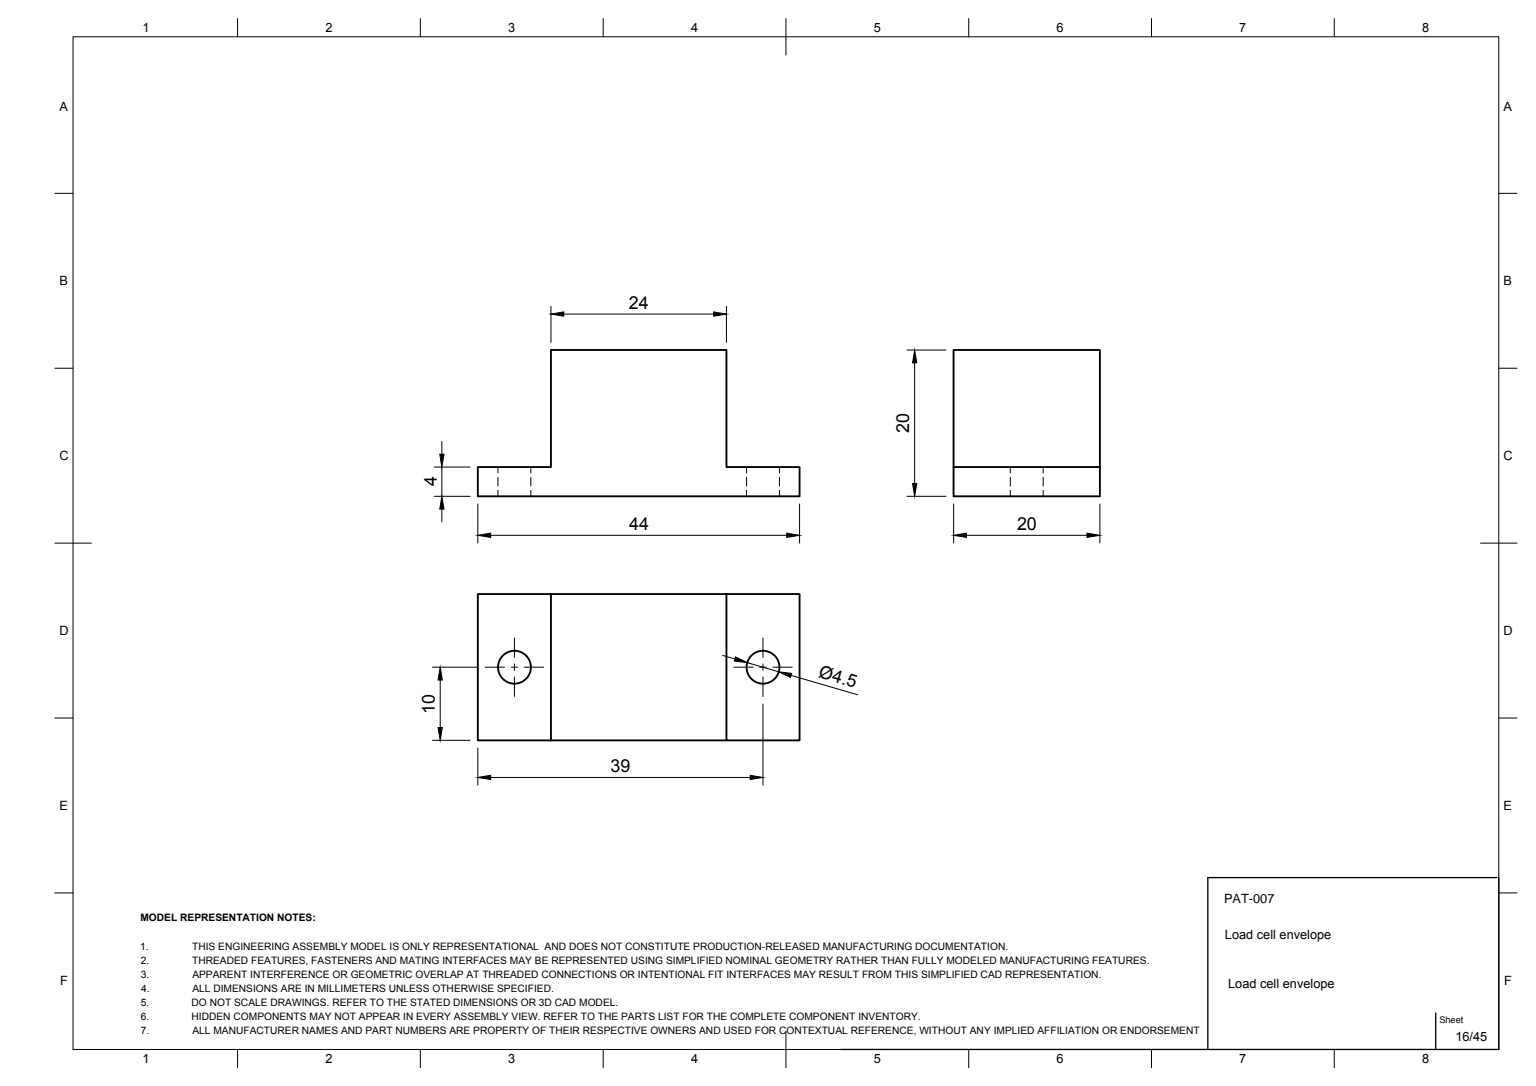
ISO-10303-21;
HEADER;
/* Generated by software containing ST-Developer
 * from STEP Tools, Inc. (www.steptools.com) 
 */

FILE_DESCRIPTION(
/* description */ ('Bearing friction torque test rig'),
/* implementation_level */ '2;1');

FILE_NAME(
/* name */ 'Load cell envelope.step',
/* time_stamp */ '2026-10-28T03:24:04-07:00',
/* author */ (''),
/* organization */ (''),
/* preprocessor_version */ 'ST-DEVELOPER v20.2',
/* originating_system */ 'Autodesk Translation Framework v15.17.0.0',
/* authorisation */ '');

FILE_SCHEMA (('AUTOMOTIVE_DESIGN { 1 0 10303 214 3 1 1 }'));
ENDSEC;

DATA;
#10=MECHANICAL_DESIGN_GEOMETRIC_PRESENTATION_REPRESENTATION('',(#550),#14822);
#472=SHAPE_REPRESENTATION_RELATIONSHIP('SRR','None',#15011,#511);
#511=ADVANCED_BREP_SHAPE_REPRESENTATION('',(#604),#14791);
#550=STYLED_ITEM('',(#15270),#604);
#604=MANIFOLD_SOLID_BREP('Body1',#7666);
#791=FACE_BOUND('',#1849,.T.);
#792=FACE_BOUND('',#1853,.T.);
#793=FACE_BOUND('',#1860,.T.);
#794=FACE_BOUND('',#1861,.T.);
#939=PLANE('',#8507);
#940=PLANE('',#8508);
#941=PLANE('',#8509);
#942=PLANE('',#8510);
#943=PLANE('',#8511);
#944=PLANE('',#8512);
#945=PLANE('',#8513);
#946=PLANE('',#8514);
#947=PLANE('',#8515);
#948=PLANE('',#8516);
#1254=FACE_OUTER_BOUND('',#1846,.T.);
#1255=FACE_OUTER_BOUND('',#1847,.T.);
#1256=FACE_OUTER_BOUND('',#1848,.T.);
#1257=FACE_OUTER_BOUND('',#1850,.T.);
#1258=FACE_OUTER_BOUND('',#1851,.T.);
#1259=FACE_OUTER_BOUND('',#1852,.T.);
#1260=FACE_OUTER_BOUND('',#1854,.T.);
#1261=FACE_OUTER_BOUND('',#1855,.T.);
#1262=FACE_OUTER_BOUND('',#1856,.T.);
#1263=FACE_OUTER_BOUND('',#1857,.T.);
#1264=FACE_OUTER_BOUND('',#1858,.T.);
#1265=FACE_OUTER_BOUND('',#1859,.T.);
#1846=EDGE_LOOP('',(#5844,#5845,#5846,#5847));
#1847=EDGE_LOOP('',(#5848,#5849,#5850,#5851));
#1848=EDGE_LOOP('',(#5852,#5853,#5854,#5855));
#1849=EDGE_LOOP('',(#5856));
#1850=EDGE_LOOP('',(#5857,#5858,#5859,#5860));
#1851=EDGE_LOOP('',(#5861,#5862,#5863,#5864));
#1852=EDGE_LOOP('',(#5865,#5866,#5867,#5868));
#1853=EDGE_LOOP('',(#5869));
#1854=EDGE_LOOP('',(#5870,#5871,#5872,#5873));
#1855=EDGE_LOOP('',(#5874,#5875,#5876,#5877,#5878,#5879,#5880,#5881));
#1856=EDGE_LOOP('',(#5882,#5883,#5884,#5885));
#1857=EDGE_LOOP('',(#5886,#5887,#5888,#5889,#5890,#5891,#5892,#5893));
#1858=EDGE_LOOP('',(#5894,#5895,#5896,#5897));
#1859=EDGE_LOOP('',(#5898,#5899,#5900,#5901));
#1860=EDGE_LOOP('',(#5902));
#1861=EDGE_LOOP('',(#5903));
#2377=LINE('',#12411,#2821);
#2378=LINE('',#12417,#2822);
#2379=LINE('',#12422,#2823);
#2380=LINE('',#12424,#2824);
#2381=LINE('',#12426,#2825);
#2382=LINE('',#12427,#2826);
#2383=LINE('',#12430,#2827);
#2384=LINE('',#12432,#2828);
#2385=LINE('',#12433,#2829);
#2386=LINE('',#12436,#2830);
#2387=LINE('',#12438,#2831);
#2388=LINE('',#12439,#2832);
#2389=LINE('',#12443,#2833);
#2390=LINE('',#12445,#2834);
#2391=LINE('',#12447,#2835);
#2392=LINE('',#12448,#2836);
#2393=LINE('',#12451,#2837);
#2394=LINE('',#12453,#2838);
#2395=LINE('',#12454,#2839);
#2396=LINE('',#12456,#2840);
#2397=LINE('',#12458,#2841);
#2398=LINE('',#12459,#2842);
#2399=LINE('',#12462,#2843);
#2400=LINE('',#12463,#2844);
#2401=LINE('',#12465,#2845);
#2402=LINE('',#12466,#2846);
#2821=VECTOR('',#10046,0.225);
#2822=VECTOR('',#10053,0.225);
#2823=VECTOR('',#10058,1.);
#2824=VECTOR('',#10059,1.);
#2825=VECTOR('',#10060,1.);
#2826=VECTOR('',#10061,1.);
#2827=VECTOR('',#10064,1.);
#2828=VECTOR('',#10065,1.);
#2829=VECTOR('',#10066,1.);
#2830=VECTOR('',#10069,1.);
#2831=VECTOR('',#10070,1.);
#2832=VECTOR('',#10071,1.);
#2833=VECTOR('',#10074,1.);
#2834=VECTOR('',#10075,1.);
#2835=VECTOR('',#10076,1.);
#2836=VECTOR('',#10077,1.);
#2837=VECTOR('',#10080,1.);
#2838=VECTOR('',#10081,1.);
#2839=VECTOR('',#10082,1.);
#2840=VECTOR('',#10085,1.);
#2841=VECTOR('',#10086,1.);
#2842=VECTOR('',#10087,1.);
#2843=VECTOR('',#10090,1.);
#2844=VECTOR('',#10091,1.);
#2845=VECTOR('',#10094,1.);
#2846=VECTOR('',#10095,1.);
#3291=CIRCLE('',#8502,0.225);
#3292=CIRCLE('',#8503,0.225);
#3293=CIRCLE('',#8505,0.225);
#3294=CIRCLE('',#8506,0.225);
#3785=VERTEX_POINT('',#12408);
#3786=VERTEX_POINT('',#12410);
#3787=VERTEX_POINT('',#12414);
#3788=VERTEX_POINT('',#12416);
#3789=VERTEX_POINT('',#12420);
#3790=VERTEX_POINT('',#12421);
#3791=VERTEX_POINT('',#12423);
#3792=VERTEX_POINT('',#12425);
#3793=VERTEX_POINT('',#12429);
#3794=VERTEX_POINT('',#12431);
#3795=VERTEX_POINT('',#12435);
#3796=VERTEX_POINT('',#12437);
#3797=VERTEX_POINT('',#12441);
#3798=VERTEX_POINT('',#12442);
#3799=VERTEX_POINT('',#12444);
#3800=VERTEX_POINT('',#12446);
#3801=VERTEX_POINT('',#12450);
#3802=VERTEX_POINT('',#12452);
#3803=VERTEX_POINT('',#12457);
#3804=VERTEX_POINT('',#12461);
#4548=EDGE_CURVE('',#3785,#3785,#3291,.T.);
#4549=EDGE_CURVE('',#3785,#3786,#2377,.T.);
#4550=EDGE_CURVE('',#3786,#3786,#3292,.T.);
#4551=EDGE_CURVE('',#3787,#3787,#3293,.T.);
#4552=EDGE_CURVE('',#3787,#3788,#2378,.T.);
#4553=EDGE_CURVE('',#3788,#3788,#3294,.T.);
#4554=EDGE_CURVE('',#3789,#3790,#2379,.T.);
#4555=EDGE_CURVE('',#3789,#3791,#2380,.T.);
#4556=EDGE_CURVE('',#3792,#3791,#2381,.T.);
#4557=EDGE_CURVE('',#3790,#3792,#2382,.T.);
#4558=EDGE_CURVE('',#3791,#3793,#2383,.T.);
#4559=EDGE_CURVE('',#3793,#3794,#2384,.T.);
#4560=EDGE_CURVE('',#3794,#3792,#2385,.T.);
#4561=EDGE_CURVE('',#3790,#3795,#2386,.T.);
#4562=EDGE_CURVE('',#3796,#3795,#2387,.T.);
#4563=EDGE_CURVE('',#3789,#3796,#2388,.T.);
#4564=EDGE_CURVE('',#3797,#3798,#2389,.T.);
#4565=EDGE_CURVE('',#3797,#3799,#2390,.T.);
#4566=EDGE_CURVE('',#3800,#3799,#2391,.T.);
#4567=EDGE_CURVE('',#3798,#3800,#2392,.T.);
#4568=EDGE_CURVE('',#3798,#3801,#2393,.T.);
#4569=EDGE_CURVE('',#3801,#3802,#2394,.T.);
#4570=EDGE_CURVE('',#3802,#3797,#2395,.T.);
#4571=EDGE_CURVE('',#3802,#3793,#2396,.T.);
#4572=EDGE_CURVE('',#3803,#3796,#2397,.T.);
#4573=EDGE_CURVE('',#3799,#3803,#2398,.T.);
#4574=EDGE_CURVE('',#3804,#3803,#2399,.T.);
#4575=EDGE_CURVE('',#3800,#3804,#2400,.T.);
#4576=EDGE_CURVE('',#3794,#3801,#2401,.T.);
#4577=EDGE_CURVE('',#3795,#3804,#2402,.T.);
#5844=ORIENTED_EDGE('',*,*,#4548,.F.);
#5845=ORIENTED_EDGE('',*,*,#4549,.T.);
#5846=ORIENTED_EDGE('',*,*,#4550,.F.);
#5847=ORIENTED_EDGE('',*,*,#4549,.F.);
#5848=ORIENTED_EDGE('',*,*,#4551,.F.);
#5849=ORIENTED_EDGE('',*,*,#4552,.T.);
#5850=ORIENTED_EDGE('',*,*,#4553,.F.);
#5851=ORIENTED_EDGE('',*,*,#4552,.F.);
#5852=ORIENTED_EDGE('',*,*,#4554,.F.);
#5853=ORIENTED_EDGE('',*,*,#4555,.T.);
#5854=ORIENTED_EDGE('',*,*,#4556,.F.);
#5855=ORIENTED_EDGE('',*,*,#4557,.F.);
#5856=ORIENTED_EDGE('',*,*,#4553,.T.);
#5857=ORIENTED_EDGE('',*,*,#4556,.T.);
#5858=ORIENTED_EDGE('',*,*,#4558,.T.);
#5859=ORIENTED_EDGE('',*,*,#4559,.T.);
#5860=ORIENTED_EDGE('',*,*,#4560,.T.);
#5861=ORIENTED_EDGE('',*,*,#4554,.T.);
#5862=ORIENTED_EDGE('',*,*,#4561,.T.);
#5863=ORIENTED_EDGE('',*,*,#4562,.F.);
#5864=ORIENTED_EDGE('',*,*,#4563,.F.);
#5865=ORIENTED_EDGE('',*,*,#4564,.F.);
#5866=ORIENTED_EDGE('',*,*,#4565,.T.);
#5867=ORIENTED_EDGE('',*,*,#4566,.F.);
#5868=ORIENTED_EDGE('',*,*,#4567,.F.);
#5869=ORIENTED_EDGE('',*,*,#4550,.T.);
#5870=ORIENTED_EDGE('',*,*,#4564,.T.);
#5871=ORIENTED_EDGE('',*,*,#4568,.T.);
#5872=ORIENTED_EDGE('',*,*,#4569,.T.);
#5873=ORIENTED_EDGE('',*,*,#4570,.T.);
#5874=ORIENTED_EDGE('',*,*,#4571,.T.);
#5875=ORIENTED_EDGE('',*,*,#4558,.F.);
#5876=ORIENTED_EDGE('',*,*,#4555,.F.);
#5877=ORIENTED_EDGE('',*,*,#4563,.T.);
#5878=ORIENTED_EDGE('',*,*,#4572,.F.);
#5879=ORIENTED_EDGE('',*,*,#4573,.F.);
#5880=ORIENTED_EDGE('',*,*,#4565,.F.);
#5881=ORIENTED_EDGE('',*,*,#4570,.F.);
#5882=ORIENTED_EDGE('',*,*,#4566,.T.);
#5883=ORIENTED_EDGE('',*,*,#4573,.T.);
#5884=ORIENTED_EDGE('',*,*,#4574,.F.);
#5885=ORIENTED_EDGE('',*,*,#4575,.F.);
#5886=ORIENTED_EDGE('',*,*,#4576,.T.);
#5887=ORIENTED_EDGE('',*,*,#4568,.F.);
#5888=ORIENTED_EDGE('',*,*,#4567,.T.);
#5889=ORIENTED_EDGE('',*,*,#4575,.T.);
#5890=ORIENTED_EDGE('',*,*,#4577,.F.);
#5891=ORIENTED_EDGE('',*,*,#4561,.F.);
#5892=ORIENTED_EDGE('',*,*,#4557,.T.);
#5893=ORIENTED_EDGE('',*,*,#4560,.F.);
#5894=ORIENTED_EDGE('',*,*,#4577,.T.);
#5895=ORIENTED_EDGE('',*,*,#4574,.T.);
#5896=ORIENTED_EDGE('',*,*,#4572,.T.);
#5897=ORIENTED_EDGE('',*,*,#4562,.T.);
#5898=ORIENTED_EDGE('',*,*,#4576,.F.);
#5899=ORIENTED_EDGE('',*,*,#4559,.F.);
#5900=ORIENTED_EDGE('',*,*,#4571,.F.);
#5901=ORIENTED_EDGE('',*,*,#4569,.F.);
#5902=ORIENTED_EDGE('',*,*,#4548,.T.);
#5903=ORIENTED_EDGE('',*,*,#4551,.T.);
#7134=CYLINDRICAL_SURFACE('',#8501,0.225);
#7135=CYLINDRICAL_SURFACE('',#8504,0.225);
#7365=ADVANCED_FACE('',(#1254),#7134,.F.);
#7366=ADVANCED_FACE('',(#1255),#7135,.F.);
#7367=ADVANCED_FACE('',(#1256,#791),#939,.T.);
#7368=ADVANCED_FACE('',(#1257),#940,.T.);
#7369=ADVANCED_FACE('',(#1258),#941,.T.);
#7370=ADVANCED_FACE('',(#1259,#792),#942,.T.);
#7371=ADVANCED_FACE('',(#1260),#943,.F.);
#7372=ADVANCED_FACE('',(#1261),#944,.T.);
#7373=ADVANCED_FACE('',(#1262),#945,.T.);
#7374=ADVANCED_FACE('',(#1263),#946,.T.);
#7375=ADVANCED_FACE('',(#1264),#947,.T.);
#7376=ADVANCED_FACE('',(#1265,#793,#794),#948,.F.);
#7666=CLOSED_SHELL('',(#7365,#7366,#7367,#7368,#7369,#7370,#7371,#7372,
#7373,#7374,#7375,#7376));
#8500=AXIS2_PLACEMENT_3D('',#12406,#10040,#10041);
#8501=AXIS2_PLACEMENT_3D('',#12407,#10042,#10043);
#8502=AXIS2_PLACEMENT_3D('',#12409,#10044,#10045);
#8503=AXIS2_PLACEMENT_3D('',#12412,#10047,#10048);
#8504=AXIS2_PLACEMENT_3D('',#12413,#10049,#10050);
#8505=AXIS2_PLACEMENT_3D('',#12415,#10051,#10052);
#8506=AXIS2_PLACEMENT_3D('',#12418,#10054,#10055);
#8507=AXIS2_PLACEMENT_3D('',#12419,#10056,#10057);
#8508=AXIS2_PLACEMENT_3D('',#12428,#10062,#10063);
#8509=AXIS2_PLACEMENT_3D('',#12434,#10067,#10068);
#8510=AXIS2_PLACEMENT_3D('',#12440,#10072,#10073);
#8511=AXIS2_PLACEMENT_3D('',#12449,#10078,#10079);
#8512=AXIS2_PLACEMENT_3D('',#12455,#10083,#10084);
#8513=AXIS2_PLACEMENT_3D('',#12460,#10088,#10089);
#8514=AXIS2_PLACEMENT_3D('',#12464,#10092,#10093);
#8515=AXIS2_PLACEMENT_3D('',#12467,#10096,#10097);
#8516=AXIS2_PLACEMENT_3D('',#12468,#10098,#10099);
#10040=DIRECTION('axis',(0.,0.,1.));
#10041=DIRECTION('refdir',(1.,0.,0.));
#10042=DIRECTION('center_axis',(0.,0.,1.));
#10043=DIRECTION('ref_axis',(1.,0.,0.));
#10044=DIRECTION('center_axis',(0.,0.,1.));
#10045=DIRECTION('ref_axis',(1.,0.,0.));
#10046=DIRECTION('',(0.,0.,1.));
#10047=DIRECTION('center_axis',(0.,0.,-1.));
#10048=DIRECTION('ref_axis',(1.,0.,0.));
#10049=DIRECTION('center_axis',(0.,0.,1.));
#10050=DIRECTION('ref_axis',(1.,0.,0.));
#10051=DIRECTION('center_axis',(0.,0.,1.));
#10052=DIRECTION('ref_axis',(1.,0.,0.));
#10053=DIRECTION('',(0.,0.,1.));
#10054=DIRECTION('center_axis',(0.,0.,-1.));
#10055=DIRECTION('ref_axis',(1.,0.,0.));
#10056=DIRECTION('center_axis',(0.,0.,1.));
#10057=DIRECTION('ref_axis',(1.,0.,0.));
#10058=DIRECTION('',(-1.,0.,0.));
#10059=DIRECTION('',(0.,1.,0.));
#10060=DIRECTION('',(1.,0.,0.));
#10061=DIRECTION('',(0.,1.,0.));
#10062=DIRECTION('center_axis',(0.,1.,0.));
#10063=DIRECTION('ref_axis',(0.,0.,1.));
#10064=DIRECTION('',(0.,0.,-1.));
#10065=DIRECTION('',(-1.,0.,0.));
#10066=DIRECTION('',(0.,0.,1.));
#10067=DIRECTION('center_axis',(0.,1.,0.));
#10068=DIRECTION('ref_axis',(-1.,0.,0.));
#10069=DIRECTION('',(0.,0.,1.));
#10070=DIRECTION('',(-1.,0.,0.));
#10071=DIRECTION('',(0.,0.,1.));
#10072=DIRECTION('center_axis',(0.,0.,1.));
#10073=DIRECTION('ref_axis',(1.,0.,0.));
#10074=DIRECTION('',(-1.,0.,0.));
#10075=DIRECTION('',(0.,1.,0.));
#10076=DIRECTION('',(1.,0.,0.));
#10077=DIRECTION('',(0.,1.,0.));
#10078=DIRECTION('center_axis',(0.,1.,0.));
#10079=DIRECTION('ref_axis',(1.,0.,0.));
#10080=DIRECTION('',(0.,0.,-1.));
#10081=DIRECTION('',(1.,0.,0.));
#10082=DIRECTION('',(0.,0.,1.));
#10083=DIRECTION('center_axis',(1.,0.,0.));
#10084=DIRECTION('ref_axis',(0.,1.,0.));
#10085=DIRECTION('',(0.,1.,0.));
#10086=DIRECTION('',(0.,1.,0.));
#10087=DIRECTION('',(0.,0.,1.));
#10088=DIRECTION('center_axis',(0.,-1.,0.));
#10089=DIRECTION('ref_axis',(1.,0.,0.));
#10090=DIRECTION('',(1.,0.,0.));
#10091=DIRECTION('',(0.,0.,1.));
#10092=DIRECTION('center_axis',(-1.,0.,0.));
#10093=DIRECTION('ref_axis',(0.,-1.,0.));
#10094=DIRECTION('',(0.,-1.,0.));
#10095=DIRECTION('',(0.,-1.,0.));
#10096=DIRECTION('center_axis',(0.,0.,1.));
#10097=DIRECTION('ref_axis',(1.,0.,0.));
#10098=DIRECTION('center_axis',(0.,0.,1.));
#10099=DIRECTION('ref_axis',(1.,0.,0.));
#12406=CARTESIAN_POINT('',(0.,0.,0.));
#12407=CARTESIAN_POINT('Origin',(10.,-1.7,4.4));
#12408=CARTESIAN_POINT('',(9.775,-1.7,4.5));
#12409=CARTESIAN_POINT('Origin',(10.,-1.7,4.5));
#12410=CARTESIAN_POINT('',(9.775,-1.7,4.9));
#12411=CARTESIAN_POINT('',(9.775,-1.7,4.4));
#12412=CARTESIAN_POINT('Origin',(10.,-1.7,4.9));
#12413=CARTESIAN_POINT('Origin',(10.,1.7,4.4));
#12414=CARTESIAN_POINT('',(9.775,1.7,4.5));
#12415=CARTESIAN_POINT('Origin',(10.,1.7,4.5));
#12416=CARTESIAN_POINT('',(9.775,1.7,4.9));
#12417=CARTESIAN_POINT('',(9.775,1.7,4.4));
#12418=CARTESIAN_POINT('Origin',(10.,1.7,4.9));
#12419=CARTESIAN_POINT('Origin',(9.,1.2,4.9));
#12420=CARTESIAN_POINT('',(11.,1.2,4.9));
#12421=CARTESIAN_POINT('',(9.,1.2,4.9));
#12422=CARTESIAN_POINT('',(10.,1.2,4.9));
#12423=CARTESIAN_POINT('',(11.,2.2,4.9));
#12424=CARTESIAN_POINT('',(11.,1.2,4.9));
#12425=CARTESIAN_POINT('',(9.,2.2,4.9));
#12426=CARTESIAN_POINT('',(11.,2.2,4.9));
#12427=CARTESIAN_POINT('',(9.,1.2,4.9));
#12428=CARTESIAN_POINT('Origin',(10.,2.2,4.7));
#12429=CARTESIAN_POINT('',(11.,2.2,4.5));
#12430=CARTESIAN_POINT('',(11.,2.2,4.5));
#12431=CARTESIAN_POINT('',(9.,2.2,4.5));
#12432=CARTESIAN_POINT('',(9.,2.2,4.5));
#12433=CARTESIAN_POINT('',(9.,2.2,4.9));
#12434=CARTESIAN_POINT('Origin',(11.,1.2,4.5));
#12435=CARTESIAN_POINT('',(9.,1.2,6.5));
#12436=CARTESIAN_POINT('',(9.,1.2,4.5));
#12437=CARTESIAN_POINT('',(11.,1.2,6.5));
#12438=CARTESIAN_POINT('',(11.,1.2,6.5));
#12439=CARTESIAN_POINT('',(11.,1.2,4.5));
#12440=CARTESIAN_POINT('Origin',(9.,-2.2,4.9));
#12441=CARTESIAN_POINT('',(11.,-2.2,4.9));
#12442=CARTESIAN_POINT('',(9.,-2.2,4.9));
#12443=CARTESIAN_POINT('',(11.,-2.2,4.9));
#12444=CARTESIAN_POINT('',(11.,-1.2,4.9));
#12445=CARTESIAN_POINT('',(11.,-2.2,4.9));
#12446=CARTESIAN_POINT('',(9.,-1.2,4.9));
#12447=CARTESIAN_POINT('',(9.,-1.2,4.9));
#12448=CARTESIAN_POINT('',(9.,-2.2,4.9));
#12449=CARTESIAN_POINT('Origin',(10.,-2.2,4.7));
#12450=CARTESIAN_POINT('',(9.,-2.2,4.5));
#12451=CARTESIAN_POINT('',(9.,-2.2,4.9));
#12452=CARTESIAN_POINT('',(11.,-2.2,4.5));
#12453=CARTESIAN_POINT('',(9.,-2.2,4.5));
#12454=CARTESIAN_POINT('',(11.,-2.2,4.5));
#12455=CARTESIAN_POINT('Origin',(11.,-1.2,4.5));
#12456=CARTESIAN_POINT('',(11.,-2.2,4.5));
#12457=CARTESIAN_POINT('',(11.,-1.2,6.5));
#12458=CARTESIAN_POINT('',(11.,-1.2,6.5));
#12459=CARTESIAN_POINT('',(11.,-1.2,4.5));
#12460=CARTESIAN_POINT('Origin',(9.,-1.2,4.5));
#12461=CARTESIAN_POINT('',(9.,-1.2,6.5));
#12462=CARTESIAN_POINT('',(9.,-1.2,6.5));
#12463=CARTESIAN_POINT('',(9.,-1.2,4.5));
#12464=CARTESIAN_POINT('Origin',(9.,1.2,4.5));
#12465=CARTESIAN_POINT('',(9.,1.2,4.5));
#12466=CARTESIAN_POINT('',(9.,1.2,6.5));
#12467=CARTESIAN_POINT('Origin',(10.,0.,6.5));
#12468=CARTESIAN_POINT('Origin',(10.,0.,4.5));
#14746=UNCERTAINTY_MEASURE_WITH_UNIT(LENGTH_MEASURE(0.001),#14823,
'DISTANCE_ACCURACY_VALUE',
'Maximum model space distance between geometric entities at asserted c
onnectivities');
#14777=UNCERTAINTY_MEASURE_WITH_UNIT(LENGTH_MEASURE(0.001),#14823,
'DISTANCE_ACCURACY_VALUE',
'Maximum model space distance between geometric entities at asserted c
onnectivities');
#14791=(
GEOMETRIC_REPRESENTATION_CONTEXT(3)
GLOBAL_UNCERTAINTY_ASSIGNED_CONTEXT((#14746))
GLOBAL_UNIT_ASSIGNED_CONTEXT((#14823,#14825,#14826))
REPRESENTATION_CONTEXT('','3D')
);
#14822=(
GEOMETRIC_REPRESENTATION_CONTEXT(3)
GLOBAL_UNCERTAINTY_ASSIGNED_CONTEXT((#14777))
GLOBAL_UNIT_ASSIGNED_CONTEXT((#14823,#14825,#14826))
REPRESENTATION_CONTEXT('','3D')
);
#14823=(
LENGTH_UNIT()
NAMED_UNIT(*)
SI_UNIT(.CENTI.,.METRE.)
);
#14825=(
NAMED_UNIT(*)
PLANE_ANGLE_UNIT()
SI_UNIT($,.RADIAN.)
);
#14826=(
NAMED_UNIT(*)
SI_UNIT($,.STERADIAN.)
SOLID_ANGLE_UNIT()
);
#14840=SHAPE_DEFINITION_REPRESENTATION(#14884,#15011);
#14884=PRODUCT_DEFINITION_SHAPE('',$,#15056);
#15011=SHAPE_REPRESENTATION('',(#8500),#14791);
#15042=PRODUCT_DEFINITION_CONTEXT('part definition',#15176,'design');
#15056=PRODUCT_DEFINITION('Load cell envelope','Load cell envelope',#15100,
#15042);
#15100=PRODUCT_DEFINITION_FORMATION('',$,#15191);
#15176=APPLICATION_CONTEXT(
'Core Data for Automotive Mechanical Design Process');
#15177=PRODUCT_CONTEXT('part definition',#15176,'mechanical');
#15191=PRODUCT('Load cell envelope','Load cell envelope',
'Load cell envelope',(#15177));
#15264=COLOUR_RGB('Light Blue',0.38,0.62,0.78);
#15265=FILL_AREA_STYLE_COLOUR('',#15264);
#15266=FILL_AREA_STYLE('',(#15265));
#15267=SURFACE_STYLE_FILL_AREA(#15266);
#15268=SURFACE_SIDE_STYLE('',(#15267));
#15269=SURFACE_STYLE_USAGE(.BOTH.,#15268);
#15270=PRESENTATION_STYLE_ASSIGNMENT((#15269));
ENDSEC;
END-ISO-10303-21;
